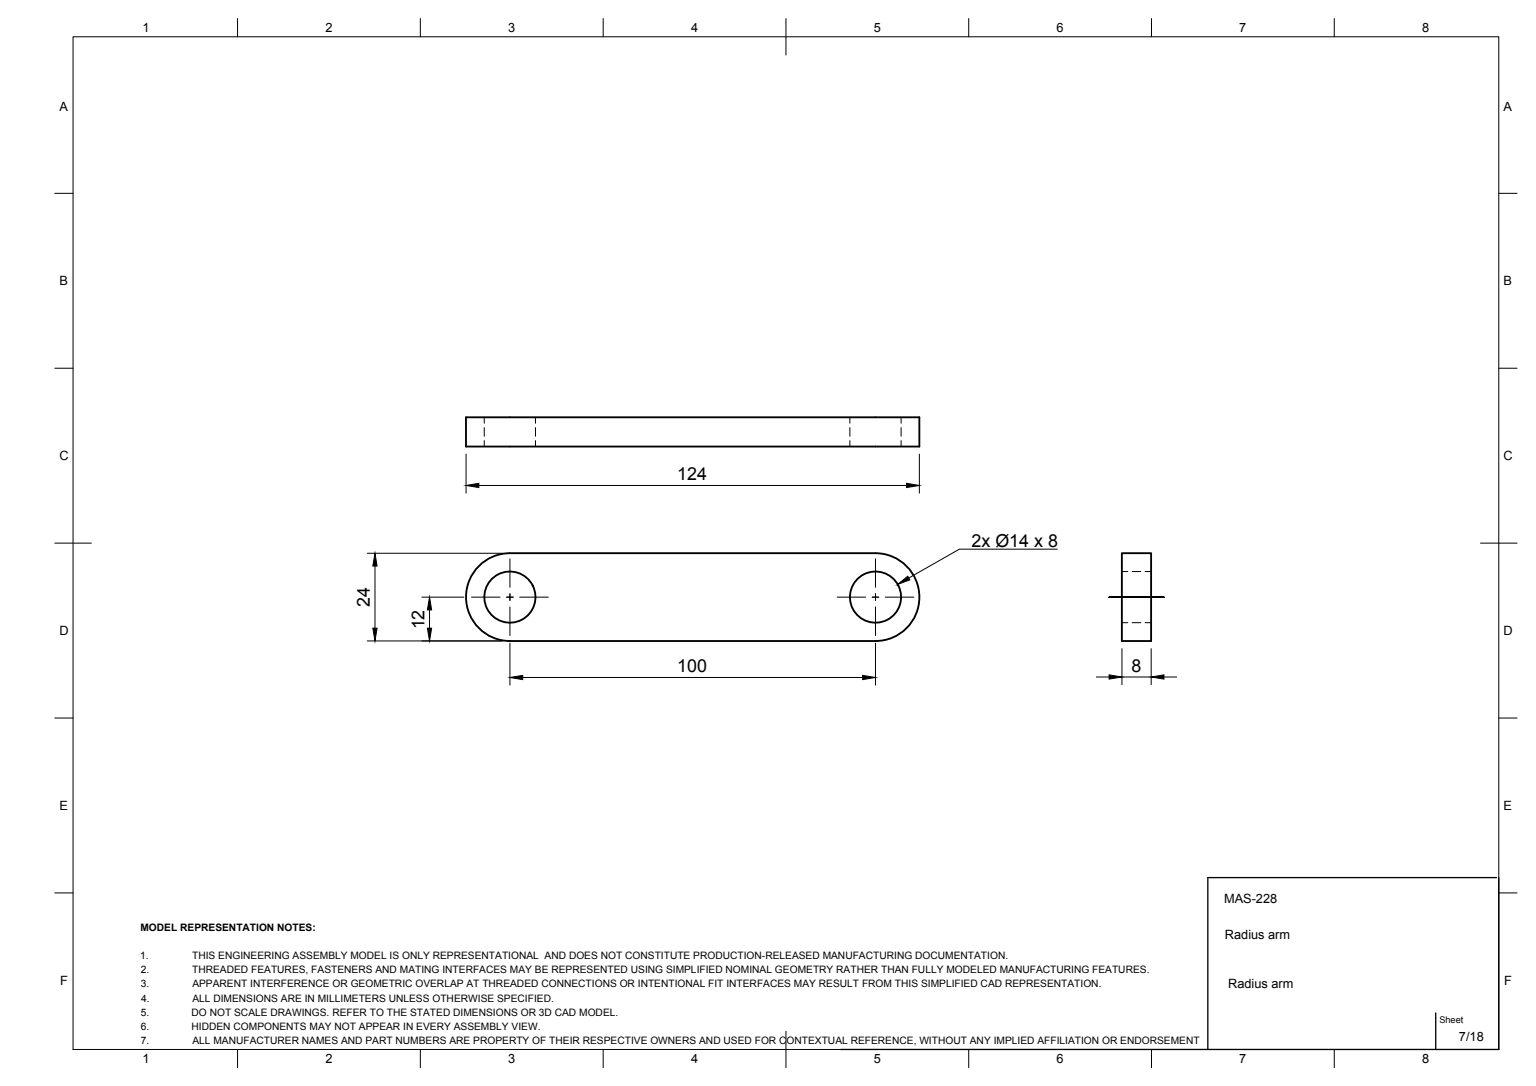
ISO-10303-21;
HEADER;
/* Generated by software containing ST-Developer
 * from STEP Tools, Inc. (www.steptools.com) 
 */

FILE_DESCRIPTION(
/* description */ ('Independent Peaucellier-Lipkin straight-line linkage. Radius arms 100
 mm, inversion-cell links 60 mm, crank radius and fixed-pivot spacing 
32 mm. Inversion constant 6400 mm squared, nominal output straight lin
e X=100 mm. Overhead bearing bridge clears the layered moving links. N
o accuracy or load rating assigned.'),
/* implementation_level */ '2;1');

FILE_NAME(
/* name */ 'Radius arm.step',
/* time_stamp */ '2026-11-09T18:06:16-08:00',
/* author */ (''),
/* organization */ (''),
/* preprocessor_version */ 'ST-DEVELOPER v20.2',
/* originating_system */ 'Autodesk Translation Framework v15.17.0.0',
/* authorisation */ '');

FILE_SCHEMA (('AUTOMOTIVE_DESIGN { 1 0 10303 214 3 1 1 }'));
ENDSEC;

DATA;
#10=MECHANICAL_DESIGN_GEOMETRIC_PRESENTATION_REPRESENTATION('',(#287),#3581);
#253=SHAPE_REPRESENTATION_RELATIONSHIP('SRR','None',#3687,#270);
#270=ADVANCED_BREP_SHAPE_REPRESENTATION('',(#304),#3569);
#287=STYLED_ITEM('',(#3780),#304);
#304=MANIFOLD_SOLID_BREP('Body1',#1873);
#334=FACE_BOUND('',#594,.T.);
#335=FACE_BOUND('',#595,.T.);
#336=FACE_BOUND('',#597,.T.);
#337=FACE_BOUND('',#598,.T.);
#384=PLANE('',#2145);
#385=PLANE('',#2149);
#386=PLANE('',#2153);
#387=PLANE('',#2154);
#458=FACE_OUTER_BOUND('',#587,.T.);
#459=FACE_OUTER_BOUND('',#588,.T.);
#460=FACE_OUTER_BOUND('',#589,.T.);
#461=FACE_OUTER_BOUND('',#590,.T.);
#462=FACE_OUTER_BOUND('',#591,.T.);
#463=FACE_OUTER_BOUND('',#592,.T.);
#464=FACE_OUTER_BOUND('',#593,.T.);
#465=FACE_OUTER_BOUND('',#596,.T.);
#587=EDGE_LOOP('',(#1454,#1455,#1456,#1457));
#588=EDGE_LOOP('',(#1458,#1459,#1460,#1461));
#589=EDGE_LOOP('',(#1462,#1463,#1464,#1465));
#590=EDGE_LOOP('',(#1466,#1467,#1468,#1469));
#591=EDGE_LOOP('',(#1470,#1471,#1472,#1473));
#592=EDGE_LOOP('',(#1474,#1475,#1476,#1477));
#593=EDGE_LOOP('',(#1478,#1479,#1480,#1481));
#594=EDGE_LOOP('',(#1482));
#595=EDGE_LOOP('',(#1483));
#596=EDGE_LOOP('',(#1484,#1485,#1486,#1487));
#597=EDGE_LOOP('',(#1488));
#598=EDGE_LOOP('',(#1489));
#738=LINE('',#3188,#836);
#739=LINE('',#3194,#837);
#740=LINE('',#3199,#838);
#741=LINE('',#3201,#839);
#742=LINE('',#3203,#840);
#743=LINE('',#3204,#841);
#744=LINE('',#3210,#842);
#745=LINE('',#3213,#843);
#746=LINE('',#3215,#844);
#747=LINE('',#3216,#845);
#836=VECTOR('',#2538,7.);
#837=VECTOR('',#2545,7.);
#838=VECTOR('',#2550,10.);
#839=VECTOR('',#2551,10.);
#840=VECTOR('',#2552,10.);
#841=VECTOR('',#2553,10.);
#842=VECTOR('',#2560,10.);
#843=VECTOR('',#2563,10.);
#844=VECTOR('',#2564,10.);
#845=VECTOR('',#2565,10.);
#917=CIRCLE('',#2140,7.);
#918=CIRCLE('',#2141,7.);
#919=CIRCLE('',#2143,7.);
#920=CIRCLE('',#2144,7.);
#921=CIRCLE('',#2147,12.);
#922=CIRCLE('',#2148,12.);
#923=CIRCLE('',#2151,12.);
#924=CIRCLE('',#2152,12.);
#1035=VERTEX_POINT('',#3185);
#1036=VERTEX_POINT('',#3187);
#1037=VERTEX_POINT('',#3191);
#1038=VERTEX_POINT('',#3193);
#1039=VERTEX_POINT('',#3197);
#1040=VERTEX_POINT('',#3198);
#1041=VERTEX_POINT('',#3200);
#1042=VERTEX_POINT('',#3202);
#1043=VERTEX_POINT('',#3206);
#1044=VERTEX_POINT('',#3208);
#1045=VERTEX_POINT('',#3212);
#1046=VERTEX_POINT('',#3214);
#1189=EDGE_CURVE('',#1035,#1035,#917,.T.);
#1190=EDGE_CURVE('',#1035,#1036,#738,.T.);
#1191=EDGE_CURVE('',#1036,#1036,#918,.T.);
#1192=EDGE_CURVE('',#1037,#1037,#919,.T.);
#1193=EDGE_CURVE('',#1037,#1038,#739,.T.);
#1194=EDGE_CURVE('',#1038,#1038,#920,.T.);
#1195=EDGE_CURVE('',#1039,#1040,#740,.T.);
#1196=EDGE_CURVE('',#1040,#1041,#741,.T.);
#1197=EDGE_CURVE('',#1042,#1041,#742,.T.);
#1198=EDGE_CURVE('',#1039,#1042,#743,.T.);
#1199=EDGE_CURVE('',#1043,#1039,#921,.T.);
#1200=EDGE_CURVE('',#1044,#1042,#922,.T.);
#1201=EDGE_CURVE('',#1043,#1044,#744,.T.);
#1202=EDGE_CURVE('',#1045,#1043,#745,.T.);
#1203=EDGE_CURVE('',#1046,#1044,#746,.T.);
#1204=EDGE_CURVE('',#1045,#1046,#747,.T.);
#1205=EDGE_CURVE('',#1040,#1045,#923,.T.);
#1206=EDGE_CURVE('',#1041,#1046,#924,.T.);
#1454=ORIENTED_EDGE('',*,*,#1189,.F.);
#1455=ORIENTED_EDGE('',*,*,#1190,.T.);
#1456=ORIENTED_EDGE('',*,*,#1191,.F.);
#1457=ORIENTED_EDGE('',*,*,#1190,.F.);
#1458=ORIENTED_EDGE('',*,*,#1192,.F.);
#1459=ORIENTED_EDGE('',*,*,#1193,.T.);
#1460=ORIENTED_EDGE('',*,*,#1194,.F.);
#1461=ORIENTED_EDGE('',*,*,#1193,.F.);
#1462=ORIENTED_EDGE('',*,*,#1195,.T.);
#1463=ORIENTED_EDGE('',*,*,#1196,.T.);
#1464=ORIENTED_EDGE('',*,*,#1197,.F.);
#1465=ORIENTED_EDGE('',*,*,#1198,.F.);
#1466=ORIENTED_EDGE('',*,*,#1199,.T.);
#1467=ORIENTED_EDGE('',*,*,#1198,.T.);
#1468=ORIENTED_EDGE('',*,*,#1200,.F.);
#1469=ORIENTED_EDGE('',*,*,#1201,.F.);
#1470=ORIENTED_EDGE('',*,*,#1202,.T.);
#1471=ORIENTED_EDGE('',*,*,#1201,.T.);
#1472=ORIENTED_EDGE('',*,*,#1203,.F.);
#1473=ORIENTED_EDGE('',*,*,#1204,.F.);
#1474=ORIENTED_EDGE('',*,*,#1205,.T.);
#1475=ORIENTED_EDGE('',*,*,#1204,.T.);
#1476=ORIENTED_EDGE('',*,*,#1206,.F.);
#1477=ORIENTED_EDGE('',*,*,#1196,.F.);
#1478=ORIENTED_EDGE('',*,*,#1206,.T.);
#1479=ORIENTED_EDGE('',*,*,#1203,.T.);
#1480=ORIENTED_EDGE('',*,*,#1200,.T.);
#1481=ORIENTED_EDGE('',*,*,#1197,.T.);
#1482=ORIENTED_EDGE('',*,*,#1189,.T.);
#1483=ORIENTED_EDGE('',*,*,#1192,.T.);
#1484=ORIENTED_EDGE('',*,*,#1205,.F.);
#1485=ORIENTED_EDGE('',*,*,#1195,.F.);
#1486=ORIENTED_EDGE('',*,*,#1199,.F.);
#1487=ORIENTED_EDGE('',*,*,#1202,.F.);
#1488=ORIENTED_EDGE('',*,*,#1191,.T.);
#1489=ORIENTED_EDGE('',*,*,#1194,.T.);
#1721=CYLINDRICAL_SURFACE('',#2139,7.);
#1722=CYLINDRICAL_SURFACE('',#2142,7.);
#1723=CYLINDRICAL_SURFACE('',#2146,12.);
#1724=CYLINDRICAL_SURFACE('',#2150,12.);
#1790=ADVANCED_FACE('',(#458),#1721,.F.);
#1791=ADVANCED_FACE('',(#459),#1722,.F.);
#1792=ADVANCED_FACE('',(#460),#384,.T.);
#1793=ADVANCED_FACE('',(#461),#1723,.T.);
#1794=ADVANCED_FACE('',(#462),#385,.T.);
#1795=ADVANCED_FACE('',(#463),#1724,.T.);
#1796=ADVANCED_FACE('',(#464,#334,#335),#386,.T.);
#1797=ADVANCED_FACE('',(#465,#336,#337),#387,.F.);
#1873=CLOSED_SHELL('',(#1790,#1791,#1792,#1793,#1794,#1795,#1796,#1797));
#2138=AXIS2_PLACEMENT_3D('',#3183,#2532,#2533);
#2139=AXIS2_PLACEMENT_3D('',#3184,#2534,#2535);
#2140=AXIS2_PLACEMENT_3D('',#3186,#2536,#2537);
#2141=AXIS2_PLACEMENT_3D('',#3189,#2539,#2540);
#2142=AXIS2_PLACEMENT_3D('',#3190,#2541,#2542);
#2143=AXIS2_PLACEMENT_3D('',#3192,#2543,#2544);
#2144=AXIS2_PLACEMENT_3D('',#3195,#2546,#2547);
#2145=AXIS2_PLACEMENT_3D('',#3196,#2548,#2549);
#2146=AXIS2_PLACEMENT_3D('',#3205,#2554,#2555);
#2147=AXIS2_PLACEMENT_3D('',#3207,#2556,#2557);
#2148=AXIS2_PLACEMENT_3D('',#3209,#2558,#2559);
#2149=AXIS2_PLACEMENT_3D('',#3211,#2561,#2562);
#2150=AXIS2_PLACEMENT_3D('',#3217,#2566,#2567);
#2151=AXIS2_PLACEMENT_3D('',#3218,#2568,#2569);
#2152=AXIS2_PLACEMENT_3D('',#3219,#2570,#2571);
#2153=AXIS2_PLACEMENT_3D('',#3220,#2572,#2573);
#2154=AXIS2_PLACEMENT_3D('',#3221,#2574,#2575);
#2532=DIRECTION('axis',(0.,0.,1.));
#2533=DIRECTION('refdir',(1.,0.,0.));
#2534=DIRECTION('center_axis',(0.,0.,-1.));
#2535=DIRECTION('ref_axis',(1.,0.,0.));
#2536=DIRECTION('center_axis',(0.,0.,-1.));
#2537=DIRECTION('ref_axis',(1.,0.,0.));
#2538=DIRECTION('',(0.,0.,-1.));
#2539=DIRECTION('center_axis',(0.,0.,1.));
#2540=DIRECTION('ref_axis',(1.,0.,0.));
#2541=DIRECTION('center_axis',(0.,0.,-1.));
#2542=DIRECTION('ref_axis',(1.,0.,0.));
#2543=DIRECTION('center_axis',(0.,0.,-1.));
#2544=DIRECTION('ref_axis',(1.,0.,0.));
#2545=DIRECTION('',(0.,0.,-1.));
#2546=DIRECTION('center_axis',(0.,0.,1.));
#2547=DIRECTION('ref_axis',(1.,0.,0.));
#2548=DIRECTION('center_axis',(0.,1.,0.));
#2549=DIRECTION('ref_axis',(-1.,0.,0.));
#2550=DIRECTION('',(-1.,0.,0.));
#2551=DIRECTION('',(0.,0.,1.));
#2552=DIRECTION('',(-1.,0.,0.));
#2553=DIRECTION('',(0.,0.,1.));
#2554=DIRECTION('center_axis',(0.,0.,1.));
#2555=DIRECTION('ref_axis',(0.,-1.,0.));
#2556=DIRECTION('center_axis',(0.,0.,1.));
#2557=DIRECTION('ref_axis',(0.,-1.,0.));
#2558=DIRECTION('center_axis',(0.,0.,1.));
#2559=DIRECTION('ref_axis',(0.,-1.,0.));
#2560=DIRECTION('',(0.,0.,1.));
#2561=DIRECTION('center_axis',(0.,-1.,0.));
#2562=DIRECTION('ref_axis',(1.,0.,0.));
#2563=DIRECTION('',(1.,0.,0.));
#2564=DIRECTION('',(1.,0.,0.));
#2565=DIRECTION('',(0.,0.,1.));
#2566=DIRECTION('center_axis',(0.,0.,1.));
#2567=DIRECTION('ref_axis',(0.,1.,0.));
#2568=DIRECTION('center_axis',(0.,0.,1.));
#2569=DIRECTION('ref_axis',(0.,1.,0.));
#2570=DIRECTION('center_axis',(0.,0.,1.));
#2571=DIRECTION('ref_axis',(0.,1.,0.));
#2572=DIRECTION('center_axis',(0.,0.,1.));
#2573=DIRECTION('ref_axis',(1.,0.,0.));
#2574=DIRECTION('center_axis',(0.,0.,1.));
#2575=DIRECTION('ref_axis',(1.,0.,0.));
#3183=CARTESIAN_POINT('',(0.,0.,0.));
#3184=CARTESIAN_POINT('Origin',(0.,0.,4.));
#3185=CARTESIAN_POINT('',(-7.,8.57252759403147E-16,8.));
#3186=CARTESIAN_POINT('Origin',(0.,0.,8.));
#3187=CARTESIAN_POINT('',(-7.,8.57252759403147E-16,0.));
#3188=CARTESIAN_POINT('',(-7.,8.57252759403147E-16,4.));
#3189=CARTESIAN_POINT('Origin',(0.,0.,0.));
#3190=CARTESIAN_POINT('Origin',(100.,0.,4.));
#3191=CARTESIAN_POINT('',(93.,8.57252759403147E-16,8.));
#3192=CARTESIAN_POINT('Origin',(100.,0.,8.));
#3193=CARTESIAN_POINT('',(93.,8.57252759403147E-16,0.));
#3194=CARTESIAN_POINT('',(93.,8.57252759403147E-16,4.));
#3195=CARTESIAN_POINT('Origin',(100.,0.,0.));
#3196=CARTESIAN_POINT('Origin',(100.,12.,0.));
#3197=CARTESIAN_POINT('',(100.,12.,0.));
#3198=CARTESIAN_POINT('',(0.,12.,0.));
#3199=CARTESIAN_POINT('',(100.,12.,0.));
#3200=CARTESIAN_POINT('',(0.,12.,8.));
#3201=CARTESIAN_POINT('',(0.,12.,0.));
#3202=CARTESIAN_POINT('',(100.,12.,8.));
#3203=CARTESIAN_POINT('',(100.,12.,8.));
#3204=CARTESIAN_POINT('',(100.,12.,0.));
#3205=CARTESIAN_POINT('Origin',(100.,-1.11022302462516E-15,0.));
#3206=CARTESIAN_POINT('',(100.,-12.,0.));
#3207=CARTESIAN_POINT('Origin',(100.,-1.11022302462516E-15,0.));
#3208=CARTESIAN_POINT('',(100.,-12.,8.));
#3209=CARTESIAN_POINT('Origin',(100.,-1.11022302462516E-15,8.));
#3210=CARTESIAN_POINT('',(100.,-12.,0.));
#3211=CARTESIAN_POINT('Origin',(0.,-12.,0.));
#3212=CARTESIAN_POINT('',(-1.46957615897682E-15,-12.,0.));
#3213=CARTESIAN_POINT('',(0.,-12.,0.));
#3214=CARTESIAN_POINT('',(-1.46957615897682E-15,-12.,8.));
#3215=CARTESIAN_POINT('',(0.,-12.,8.));
#3216=CARTESIAN_POINT('',(-1.46957615897682E-15,-12.,0.));
#3217=CARTESIAN_POINT('Origin',(0.,0.,0.));
#3218=CARTESIAN_POINT('Origin',(0.,0.,0.));
#3219=CARTESIAN_POINT('Origin',(0.,0.,8.));
#3220=CARTESIAN_POINT('Origin',(50.,0.,8.));
#3221=CARTESIAN_POINT('Origin',(50.,0.,0.));
#3550=UNCERTAINTY_MEASURE_WITH_UNIT(LENGTH_MEASURE(0.01),#3582,
'DISTANCE_ACCURACY_VALUE',
'Maximum model space distance between geometric entities at asserted c
onnectivities');
#3562=UNCERTAINTY_MEASURE_WITH_UNIT(LENGTH_MEASURE(0.01),#3582,
'DISTANCE_ACCURACY_VALUE',
'Maximum model space distance between geometric entities at asserted c
onnectivities');
#3569=(
GEOMETRIC_REPRESENTATION_CONTEXT(3)
GLOBAL_UNCERTAINTY_ASSIGNED_CONTEXT((#3550))
GLOBAL_UNIT_ASSIGNED_CONTEXT((#3582,#3584,#3585))
REPRESENTATION_CONTEXT('','3D')
);
#3581=(
GEOMETRIC_REPRESENTATION_CONTEXT(3)
GLOBAL_UNCERTAINTY_ASSIGNED_CONTEXT((#3562))
GLOBAL_UNIT_ASSIGNED_CONTEXT((#3582,#3584,#3585))
REPRESENTATION_CONTEXT('','3D')
);
#3582=(
LENGTH_UNIT()
NAMED_UNIT(*)
SI_UNIT(.MILLI.,.METRE.)
);
#3584=(
NAMED_UNIT(*)
PLANE_ANGLE_UNIT()
SI_UNIT($,.RADIAN.)
);
#3585=(
NAMED_UNIT(*)
SI_UNIT($,.STERADIAN.)
SOLID_ANGLE_UNIT()
);
#3592=SHAPE_DEFINITION_REPRESENTATION(#3610,#3687);
#3610=PRODUCT_DEFINITION_SHAPE('',$,#3706);
#3687=SHAPE_REPRESENTATION('',(#2138),#3569);
#3699=PRODUCT_DEFINITION_CONTEXT('part definition',#3755,'design');
#3706=PRODUCT_DEFINITION('Radius arm','Radius arm',#3724,#3699);
#3724=PRODUCT_DEFINITION_FORMATION('',$,#3763);
#3755=APPLICATION_CONTEXT(
'Core Data for Automotive Mechanical Design Process');
#3756=PRODUCT_CONTEXT('part definition',#3755,'mechanical');
#3763=PRODUCT('Radius arm','Radius arm',$,(#3756));
#3780=PRESENTATION_STYLE_ASSIGNMENT((#3793));
#3793=SURFACE_STYLE_USAGE(.BOTH.,#3806);
#3806=SURFACE_SIDE_STYLE('',(#3819));
#3819=SURFACE_STYLE_FILL_AREA(#3832);
#3832=FILL_AREA_STYLE('Radius arm finish',(#3845));
#3845=FILL_AREA_STYLE_COLOUR('Radius arm finish',#3858);
#3858=COLOUR_RGB('Radius arm finish',0.0901960784313725,0.270588235294118,
0.513725490196078);
ENDSEC;
END-ISO-10303-21;
